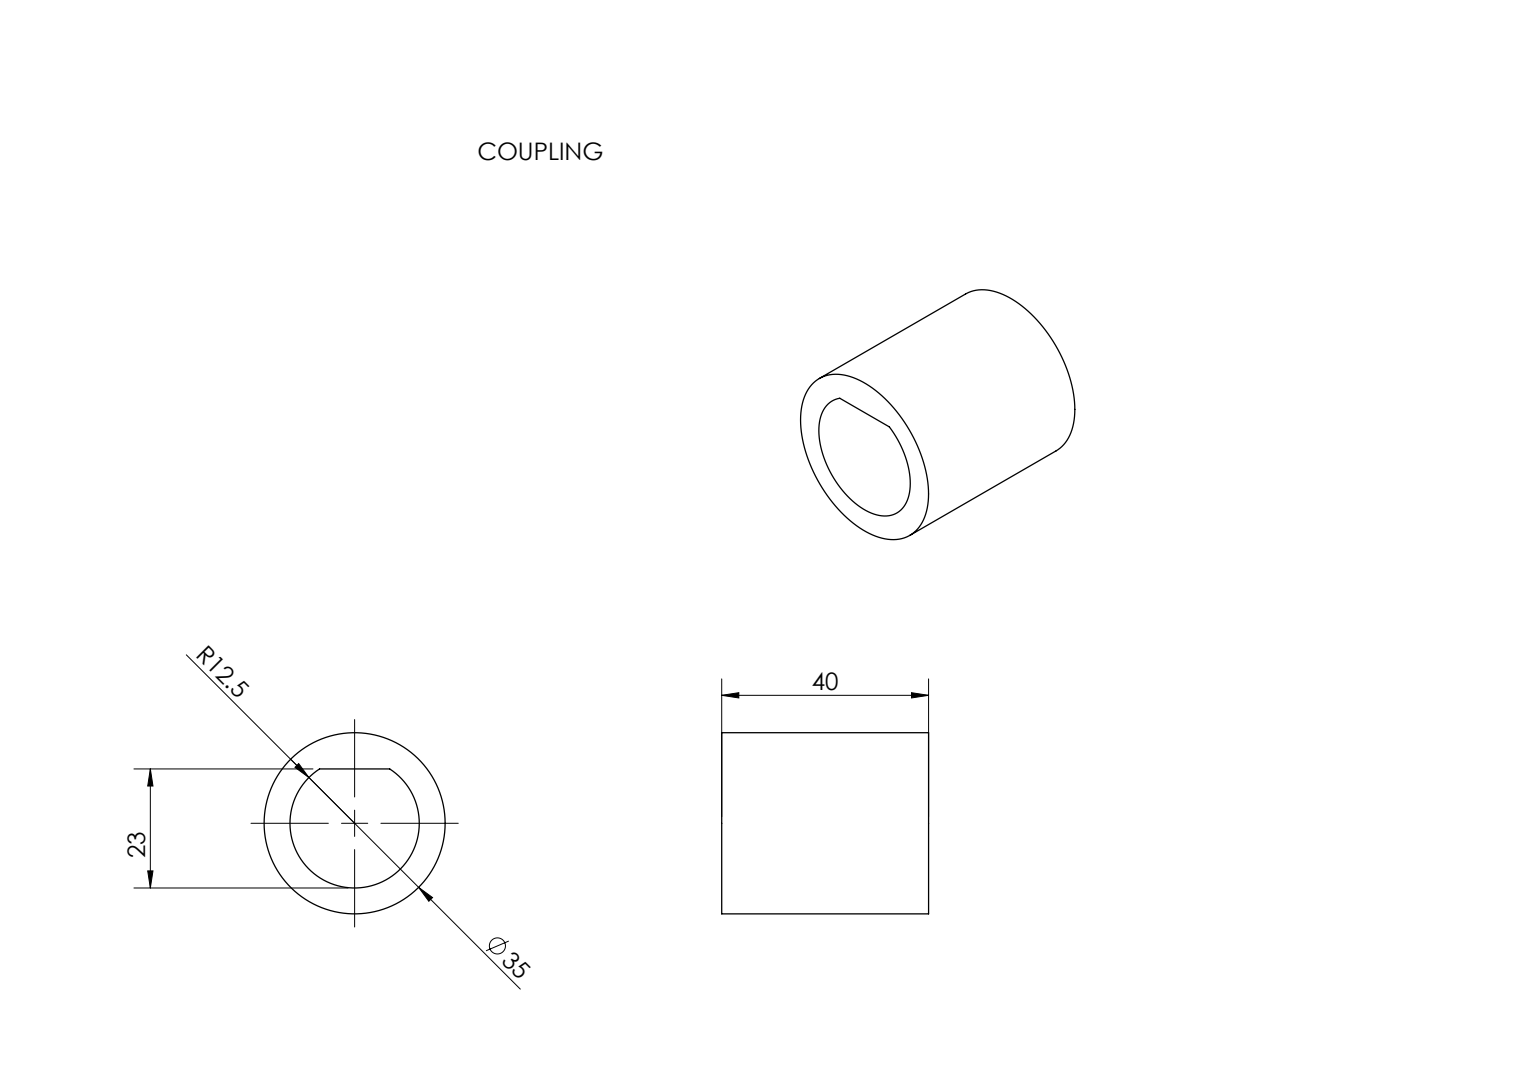
ISO-10303-21;
HEADER;
FILE_DESCRIPTION (('STEP AP214'),
    '1' );
FILE_NAME ('coupling.step',
    '2026-10-08T09:53:37',
    ( '' ),
    ( '' ),
    'SwSTEP 2.0',
    'SolidWorks 2026',
    '' );
FILE_SCHEMA (( 'AUTOMOTIVE_DESIGN' ));
ENDSEC;

DATA;
#136=DIRECTION ( 'NONE',  ( -0.000000000000000000, -0.000000000000000000, -1.000000000000000000 ) ) ;
#689=ORIENTED_EDGE ( 'NONE', *, *, #8488, .T. ) ;
#1357=DIRECTION ( 'NONE',  ( -1.000000000000000000, 0.000000000000000000, 0.000000000000000000 ) ) ;
#1430=AXIS2_PLACEMENT_3D ( 'NONE', #4521, #4148, #32316 ) ;
#1854=EDGE_CURVE ( 'NONE', #52969, #23763, #14079, .T. ) ;
#2181=EDGE_CURVE ( 'NONE', #37253, #52969, #24207, .T. ) ;
#2286=ORIENTED_EDGE ( 'NONE', *, *, #39127, .F. ) ;
#2309=UNCERTAINTY_MEASURE_WITH_UNIT (LENGTH_MEASURE( 1.000000000000000082E-05 ), #36000, 'distance_accuracy_value', 'NONE');
#2430=DIRECTION ( 'NONE',  ( 0.000000000000000000, -1.000000000000000000, 0.000000000000000000 ) ) ;
#2883=FACE_BOUND ( 'NONE', #6394, .T. ) ;
#3015=CARTESIAN_POINT ( 'NONE',  ( 12.49999999999999645, 1.530808498934191127E-15, 20.00000000000000000 ) ) ;
#3992=PRODUCT_DEFINITION_FORMATION_WITH_SPECIFIED_SOURCE ( 'ANY', '', #50605, .NOT_KNOWN. ) ;
#4148=DIRECTION ( 'NONE',  ( 0.000000000000000000, 0.000000000000000000, 1.000000000000000000 ) ) ;
#4234=CIRCLE ( 'NONE', #64274, 12.49999999999999645 ) ;
#4392=DIRECTION ( 'NONE',  ( -1.000000000000000000, 0.000000000000000000, 0.000000000000000000 ) ) ;
#4453=ORIENTED_EDGE ( 'NONE', *, *, #65373, .F. ) ;
#4521=CARTESIAN_POINT ( 'NONE',  ( 0.000000000000000000, 0.000000000000000000, -20.00000000000000000 ) ) ;
#4744=ORIENTED_EDGE ( 'NONE', *, *, #8488, .F. ) ;
#5000=ORIENTED_EDGE ( 'NONE', *, *, #5384, .T. ) ;
#5245=DIRECTION ( 'NONE',  ( 0.000000000000000000, 0.000000000000000000, 1.000000000000000000 ) ) ;
#5273=CARTESIAN_POINT ( 'NONE',  ( -12.49999999999999645, 0.000000000000000000, -20.00000000000000000 ) ) ;
#5384=EDGE_CURVE ( 'NONE', #13441, #37581, #64335, .T. ) ;
#5466=PLANE ( 'NONE',  #40740 ) ;
#5717=CARTESIAN_POINT ( 'NONE',  ( 0.000000000000000000, 0.000000000000000000, -20.00000000000000000 ) ) ;
#6168=CARTESIAN_POINT ( 'NONE',  ( 0.000000000000000000, 0.000000000000000000, 20.00000000000000000 ) ) ;
#6394=EDGE_LOOP ( 'NONE', ( #46540, #31405, #68145, #19160 ) ) ;
#6936=CARTESIAN_POINT ( 'NONE',  ( 6.782329983125270800, 10.49999999999999467, -20.00000000000000000 ) ) ;
#7059=( NAMED_UNIT ( * ) PLANE_ANGLE_UNIT ( ) SI_UNIT ( $, .RADIAN. ) );
#7688=DIRECTION ( 'NONE',  ( 0.000000000000000000, 0.000000000000000000, 1.000000000000000000 ) ) ;
#8488=EDGE_CURVE ( 'NONE', #35321, #37581, #20662, .T. ) ;
#8519=( NAMED_UNIT ( * ) PLANE_ANGLE_UNIT ( ) SI_UNIT ( $, .RADIAN. ) );
#8550=SURFACE_STYLE_FILL_AREA ( #14172 ) ;
#8566=PRODUCT_DEFINITION_CONTEXT ( 'detailed design', #29179, 'design' ) ;
#9214=VECTOR ( 'NONE', #34197, 1000.000000000000000 ) ;
#9241=SHAPE_REPRESENTATION_RELATIONSHIP ( 'NONE' , 'NONE' ,  #15311, #51651 ) ;
#9354=LINE ( 'NONE', #3015, #52898 ) ;
#9498=CARTESIAN_POINT ( 'NONE',  ( 17.50000000000000355, 2.143131898507868643E-15, -20.00000000000000000 ) ) ;
#10144=EDGE_LOOP ( 'NONE', ( #74260, #42905, #52448, #15659 ) ) ;
#10158=AXIS2_PLACEMENT_3D ( 'NONE', #38066, #2430, #54622 ) ;
#10592=CARTESIAN_POINT ( 'NONE',  ( -17.50000000000000355, 0.000000000000000000, 20.00000000000000000 ) ) ;
#11087=DIRECTION ( 'NONE',  ( 0.000000000000000000, 0.000000000000000000, 1.000000000000000000 ) ) ;
#11135=CARTESIAN_POINT ( 'NONE',  ( 0.000000000000000000, 0.000000000000000000, 20.00000000000000000 ) ) ;
#11356=CYLINDRICAL_SURFACE ( 'NONE', #17854, 17.50000000000000355 ) ;
#11556=CARTESIAN_POINT ( 'NONE',  ( 0.000000000000000000, 0.000000000000000000, -20.00000000000000000 ) ) ;
#11695=MECHANICAL_DESIGN_GEOMETRIC_PRESENTATION_REPRESENTATION('',(#51307),#56094);
#12292=VECTOR ( 'NONE', #1357, 1000.000000000000000 ) ;
#12581=LINE ( 'NONE', #6936, #12292 ) ;
#13271=DIRECTION ( 'NONE',  ( -0.000000000000000000, -0.000000000000000000, -1.000000000000000000 ) ) ;
#13441=VERTEX_POINT ( 'NONE', #51685 ) ;
#14079=CIRCLE ( 'NONE', #27275, 12.49999999999999645 ) ;
#14132=SURFACE_STYLE_FILL_AREA ( #20897 ) ;
#14172=FILL_AREA_STYLE ('',( #25830 ) ) ;
#14241=EDGE_CURVE ( 'NONE', #69413, #40595, #58506, .T. ) ;
#14507=ORIENTED_EDGE ( 'NONE', *, *, #41446, .T. ) ;
#14512=FILL_AREA_STYLE_COLOUR ( '', #15948 ) ;
#15189=DIRECTION ( 'NONE',  ( 1.000000000000000000, 0.000000000000000000, 0.000000000000000000 ) ) ;
#15190=ORIENTED_EDGE ( 'NONE', *, *, #23134, .F. ) ;
#15311=SHAPE_REPRESENTATION ( 'coupling', ( #43395 ), #59156 ) ;
#15659=ORIENTED_EDGE ( 'NONE', *, *, #38084, .F. ) ;
#15948=COLOUR_RGB ( '', 0.40784314, 0.44705882, 0.49803922) ;
#16090=EDGE_LOOP ( 'NONE', ( #39134, #689, #64984, #22017 ) ) ;
#16178=CARTESIAN_POINT ( 'NONE',  ( 0.000000000000000000, 0.000000000000000000, 20.00000000000000000 ) ) ;
#16945=ORIENTED_EDGE ( 'NONE', *, *, #47875, .T. ) ;
#16966=DIRECTION ( 'NONE',  ( 0.000000000000000000, 0.000000000000000000, 1.000000000000000000 ) ) ;
#17101=CARTESIAN_POINT ( 'NONE',  ( 0.000000000000000000, 0.000000000000000000, 20.00000000000000000 ) ) ;
#17137=MECHANICAL_DESIGN_GEOMETRIC_PRESENTATION_REPRESENTATION('',(#63986),#41183);
#17739=ORIENTED_EDGE ( 'NONE', *, *, #17822, .T. ) ;
#17822=EDGE_CURVE ( 'NONE', #50481, #37253, #39969, .T. ) ;
#17854=AXIS2_PLACEMENT_3D ( 'NONE', #45962, #136, #69617 ) ;
#17911=CIRCLE ( 'NONE', #59945, 12.49999999999999645 ) ;
#18920=ORIENTED_EDGE ( 'NONE', *, *, #2181, .T. ) ;
#19160=ORIENTED_EDGE ( 'NONE', *, *, #41446, .F. ) ;
#19592=EDGE_LOOP ( 'NONE', ( #15190, #2286, #16945, #17739 ) ) ;
#19735=DIRECTION ( 'NONE',  ( 1.000000000000000000, 0.000000000000000000, 0.000000000000000000 ) ) ;
#20145=( NAMED_UNIT ( * ) PLANE_ANGLE_UNIT ( ) SI_UNIT ( $, .RADIAN. ) );
#20557=FACE_OUTER_BOUND ( 'NONE', #10144, .T. ) ;
#20662=LINE ( 'NONE', #21020, #30170 ) ;
#20831=DIRECTION ( 'NONE',  ( -1.000000000000000000, 0.000000000000000000, 0.000000000000000000 ) ) ;
#20897=FILL_AREA_STYLE ('',( #14512 ) ) ;
#21020=CARTESIAN_POINT ( 'NONE',  ( 17.50000000000000355, 2.143131898507868643E-15, 20.00000000000000000 ) ) ;
#21820=DIRECTION ( 'NONE',  ( 0.000000000000000000, 0.000000000000000000, 1.000000000000000000 ) ) ;
#22017=ORIENTED_EDGE ( 'NONE', *, *, #42840, .F. ) ;
#22325=EDGE_LOOP ( 'NONE', ( #14507, #71175, #36244, #38954 ) ) ;
#22868=CARTESIAN_POINT ( 'NONE',  ( 6.782329983125270800, 10.49999999999999467, 20.00000000000000000 ) ) ;
#22943=EDGE_LOOP ( 'NONE', ( #18920, #29406, #40702, #64202 ) ) ;
#23134=EDGE_CURVE ( 'NONE', #68521, #37253, #12581, .T. ) ;
#23232=DIRECTION ( 'NONE',  ( 1.000000000000000000, 0.000000000000000000, 0.000000000000000000 ) ) ;
#23733=DIRECTION ( 'NONE',  ( 1.000000000000000000, 0.000000000000000000, 0.000000000000000000 ) ) ;
#23763=VERTEX_POINT ( 'NONE', #26423 ) ;
#24207=CIRCLE ( 'NONE', #1430, 12.49999999999999645 ) ;
#24681=PRODUCT_DEFINITION ( 'UNKNOWN', '', #3992, #8566 ) ;
#24741=CARTESIAN_POINT ( 'NONE',  ( 17.50000000000000355, 2.143131898507868643E-15, 20.00000000000000000 ) ) ;
#24976=FACE_OUTER_BOUND ( 'NONE', #50753, .T. ) ;
#25065=CYLINDRICAL_SURFACE ( 'NONE', #40729, 12.49999999999999645 ) ;
#25830=FILL_AREA_STYLE_COLOUR ( '', #40536 ) ;
#26093=AXIS2_PLACEMENT_3D ( 'NONE', #16178, #21820, #27829 ) ;
#26277=FACE_OUTER_BOUND ( 'NONE', #52222, .T. ) ;
#26423=CARTESIAN_POINT ( 'NONE',  ( 12.49999999999999645, 1.530808498934191127E-15, -20.00000000000000000 ) ) ;
#26883=EDGE_LOOP ( 'NONE', ( #4453, #55914, #65318, #59276 ) ) ;
#27219=AXIS2_PLACEMENT_3D ( 'NONE', #70449, #7688, #41531 ) ;
#27275=AXIS2_PLACEMENT_3D ( 'NONE', #5717, #73738, #28621 ) ;
#27829=DIRECTION ( 'NONE',  ( 1.000000000000000000, 0.000000000000000000, 0.000000000000000000 ) ) ;
#28315=LINE ( 'NONE', #72331, #38568 ) ;
#28355=ADVANCED_FACE ( 'NONE', ( #68573 ), #62952, .F. ) ;
#28616=AXIS2_PLACEMENT_3D ( 'NONE', #6168, #40735, #46010 ) ;
#28621=DIRECTION ( 'NONE',  ( 1.000000000000000000, 0.000000000000000000, 0.000000000000000000 ) ) ;
#29179=APPLICATION_CONTEXT ( 'automotive_design' ) ;
#29406=ORIENTED_EDGE ( 'NONE', *, *, #1854, .T. ) ;
#29536=CIRCLE ( 'NONE', #63221, 17.50000000000000355 ) ;
#30170=VECTOR ( 'NONE', #62009, 1000.000000000000000 ) ;
#30186=CARTESIAN_POINT ( 'NONE',  ( -17.50000000000000355, 0.000000000000000000, 20.00000000000000000 ) ) ;
#30547=AXIS2_PLACEMENT_3D ( 'NONE', #39933, #34271, #23733 ) ;
#30679=ORIENTED_EDGE ( 'NONE', *, *, #42840, .T. ) ;
#31405=ORIENTED_EDGE ( 'NONE', *, *, #14241, .F. ) ;
#31438=CARTESIAN_POINT ( 'NONE',  ( 6.782329983125270800, 10.49999999999999467, -20.00000000000000000 ) ) ;
#31919=DIRECTION ( 'NONE',  ( -1.000000000000000000, 0.000000000000000000, 0.000000000000000000 ) ) ;
#32136=ADVANCED_FACE ( 'NONE', ( #54359, #2883 ), #5466, .T. ) ;
#32188=CARTESIAN_POINT ( 'NONE',  ( 0.000000000000000000, 0.000000000000000000, 20.00000000000000000 ) ) ;
#32316=DIRECTION ( 'NONE',  ( 1.000000000000000000, 0.000000000000000000, 0.000000000000000000 ) ) ;
#32777=ADVANCED_FACE ( 'NONE', ( #51949 ), #11356, .T. ) ;
#34060=DIRECTION ( 'NONE',  ( -0.000000000000000000, -0.000000000000000000, -1.000000000000000000 ) ) ;
#34197=DIRECTION ( 'NONE',  ( -0.000000000000000000, -0.000000000000000000, -1.000000000000000000 ) ) ;
#34271=DIRECTION ( 'NONE',  ( 0.000000000000000000, 0.000000000000000000, 1.000000000000000000 ) ) ;
#35321=VERTEX_POINT ( 'NONE', #24741 ) ;
#35624=SURFACE_SIDE_STYLE ('',( #8550 ) ) ;
#36000=( LENGTH_UNIT ( ) NAMED_UNIT ( * ) SI_UNIT ( .MILLI., .METRE. ) );
#36192=DIRECTION ( 'NONE',  ( 1.000000000000000000, 0.000000000000000000, 0.000000000000000000 ) ) ;
#36244=ORIENTED_EDGE ( 'NONE', *, *, #2181, .F. ) ;
#36257=FACE_BOUND ( 'NONE', #22943, .T. ) ;
#36710=CARTESIAN_POINT ( 'NONE',  ( 0.000000000000000000, 0.000000000000000000, 20.00000000000000000 ) ) ;
#36733=PRODUCT_DEFINITION_SHAPE ( 'NONE', 'NONE',  #24681 ) ;
#37084=SURFACE_STYLE_USAGE ( .BOTH. , #54014 ) ;
#37111=DIRECTION ( 'NONE',  ( -0.000000000000000000, -0.000000000000000000, -1.000000000000000000 ) ) ;
#37253=VERTEX_POINT ( 'NONE', #74224 ) ;
#37581=VERTEX_POINT ( 'NONE', #9498 ) ;
#37592=CARTESIAN_POINT ( 'NONE',  ( -12.49999999999999645, 0.000000000000000000, 20.00000000000000000 ) ) ;
#38066=CARTESIAN_POINT ( 'NONE',  ( 6.782329983125270800, 10.49999999999999467, 20.00000000000000000 ) ) ;
#38084=EDGE_CURVE ( 'NONE', #49570, #52969, #62802, .T. ) ;
#38188=( LENGTH_UNIT ( ) NAMED_UNIT ( * ) SI_UNIT ( .MILLI., .METRE. ) );
#38212=CYLINDRICAL_SURFACE ( 'NONE', #71933, 12.49999999999999645 ) ;
#38321=CARTESIAN_POINT ( 'NONE',  ( 0.000000000000000000, 0.000000000000000000, 20.00000000000000000 ) ) ;
#38473=ORIENTED_EDGE ( 'NONE', *, *, #39207, .T. ) ;
#38568=VECTOR ( 'NONE', #20831, 1000.000000000000000 ) ;
#38954=ORIENTED_EDGE ( 'NONE', *, *, #17822, .F. ) ;
#39127=EDGE_CURVE ( 'NONE', #40595, #68521, #68712, .T. ) ;
#39134=ORIENTED_EDGE ( 'NONE', *, *, #66536, .F. ) ;
#39207=EDGE_CURVE ( 'NONE', #44003, #35321, #41733, .T. ) ;
#39393=CARTESIAN_POINT ( 'NONE',  ( 0.000000000000000000, 0.000000000000000000, 20.00000000000000000 ) ) ;
#39719=CYLINDRICAL_SURFACE ( 'NONE', #41983, 17.50000000000000355 ) ;
#39750=APPLICATION_CONTEXT ( 'automotive_design' ) ;
#39933=CARTESIAN_POINT ( 'NONE',  ( 0.000000000000000000, 0.000000000000000000, -20.00000000000000000 ) ) ;
#39969=LINE ( 'NONE', #62924, #71335 ) ;
#40536=COLOUR_RGB ( '', 0.40784314, 0.44705882, 0.49803922) ;
#40586=EDGE_CURVE ( 'NONE', #23763, #68521, #17911, .T. ) ;
#40595=VERTEX_POINT ( 'NONE', #22868 ) ;
#40702=ORIENTED_EDGE ( 'NONE', *, *, #40586, .T. ) ;
#40729=AXIS2_PLACEMENT_3D ( 'NONE', #36710, #42366, #46903 ) ;
#40734=DIRECTION ( 'NONE',  ( 0.000000000000000000, 0.000000000000000000, 1.000000000000000000 ) ) ;
#40735=DIRECTION ( 'NONE',  ( -0.000000000000000000, -0.000000000000000000, -1.000000000000000000 ) ) ;
#40740=AXIS2_PLACEMENT_3D ( 'NONE', #17101, #11087, #73854 ) ;
#40748=ADVANCED_FACE ( 'NONE', ( #52906 ), #25065, .F. ) ;
#40922=ADVANCED_FACE ( 'NONE', ( #20557 ), #38212, .F. ) ;
#41183=( GEOMETRIC_REPRESENTATION_CONTEXT ( 3 ) GLOBAL_UNCERTAINTY_ASSIGNED_CONTEXT ( ( #65621 ) ) GLOBAL_UNIT_ASSIGNED_CONTEXT ( ( #38188, #8519, #48726 ) ) REPRESENTATION_CONTEXT ( 'NONE', 'WORKASPACE' ) );
#41446=EDGE_CURVE ( 'NONE', #50481, #49570, #71877, .T. ) ;
#41531=DIRECTION ( 'NONE',  ( 1.000000000000000000, 0.000000000000000000, -0.000000000000000000 ) ) ;
#41733=CIRCLE ( 'NONE', #44096, 17.50000000000000355 ) ;
#41983=AXIS2_PLACEMENT_3D ( 'NONE', #11135, #34060, #31919 ) ;
#42028=PRESENTATION_STYLE_ASSIGNMENT (( #48029 ) ) ;
#42366=DIRECTION ( 'NONE',  ( -0.000000000000000000, -0.000000000000000000, -1.000000000000000000 ) ) ;
#42840=EDGE_CURVE ( 'NONE', #44003, #13441, #58775, .T. ) ;
#42905=ORIENTED_EDGE ( 'NONE', *, *, #65373, .T. ) ;
#43039=CARTESIAN_POINT ( 'NONE',  ( 0.000000000000000000, 0.000000000000000000, 20.00000000000000000 ) ) ;
#43063=UNCERTAINTY_MEASURE_WITH_UNIT (LENGTH_MEASURE( 1.000000000000000082E-05 ), #64548, 'distance_accuracy_value', 'NONE');
#43395=AXIS2_PLACEMENT_3D ( 'NONE', #48320, #71232, #19735 ) ;
#43941=AXIS2_PLACEMENT_3D ( 'NONE', #46372, #40734, #36192 ) ;
#44003=VERTEX_POINT ( 'NONE', #10592 ) ;
#44096=AXIS2_PLACEMENT_3D ( 'NONE', #39393, #55932, #67587 ) ;
#45962=CARTESIAN_POINT ( 'NONE',  ( 0.000000000000000000, 0.000000000000000000, 20.00000000000000000 ) ) ;
#46010=DIRECTION ( 'NONE',  ( -1.000000000000000000, 0.000000000000000000, 0.000000000000000000 ) ) ;
#46372=CARTESIAN_POINT ( 'NONE',  ( 0.000000000000000000, 0.000000000000000000, -20.00000000000000000 ) ) ;
#46512=VECTOR ( 'NONE', #56312, 1000.000000000000000 ) ;
#46540=ORIENTED_EDGE ( 'NONE', *, *, #47875, .F. ) ;
#46758=CARTESIAN_POINT ( 'NONE',  ( 12.49999999999999645, 1.530808498934191127E-15, 20.00000000000000000 ) ) ;
#46903=DIRECTION ( 'NONE',  ( -1.000000000000000000, 0.000000000000000000, 0.000000000000000000 ) ) ;
#47875=EDGE_CURVE ( 'NONE', #40595, #50481, #28315, .T. ) ;
#48029=SURFACE_STYLE_USAGE ( .BOTH. , #35624 ) ;
#48320=CARTESIAN_POINT ( 'NONE',  ( 0.000000000000000000, 0.000000000000000000, 0.000000000000000000 ) ) ;
#48519=ORIENTED_EDGE ( 'NONE', *, *, #52548, .F. ) ;
#48726=( NAMED_UNIT ( * ) SI_UNIT ( $, .STERADIAN. ) SOLID_ANGLE_UNIT ( ) );
#49279=EDGE_LOOP ( 'NONE', ( #38473, #65303 ) ) ;
#49570=VERTEX_POINT ( 'NONE', #37592 ) ;
#49701=FACE_OUTER_BOUND ( 'NONE', #19592, .T. ) ;
#50481=VERTEX_POINT ( 'NONE', #64881 ) ;
#50605=PRODUCT ( 'coupling', 'coupling', '', ( #67417 ) ) ;
#50753=EDGE_LOOP ( 'NONE', ( #55966, #48519 ) ) ;
#51081=DIRECTION ( 'NONE',  ( 1.000000000000000000, 0.000000000000000000, 0.000000000000000000 ) ) ;
#51307=STYLED_ITEM ( 'NONE', ( #42028 ), #61761 ) ;
#51412=DIRECTION ( 'NONE',  ( 0.000000000000000000, 0.000000000000000000, 1.000000000000000000 ) ) ;
#51651=ADVANCED_BREP_SHAPE_REPRESENTATION ( '', ( #61761, #43395 ), #59156 ) ;
#51685=CARTESIAN_POINT ( 'NONE',  ( -17.50000000000000355, 0.000000000000000000, -20.00000000000000000 ) ) ;
#51949=FACE_OUTER_BOUND ( 'NONE', #16090, .T. ) ;
#52222=EDGE_LOOP ( 'NONE', ( #4744, #64257, #30679, #5000 ) ) ;
#52448=ORIENTED_EDGE ( 'NONE', *, *, #1854, .F. ) ;
#52548=EDGE_CURVE ( 'NONE', #37581, #13441, #62998, .T. ) ;
#52575=VECTOR ( 'NONE', #13271, 1000.000000000000000 ) ;
#52898=VECTOR ( 'NONE', #66513, 1000.000000000000000 ) ;
#52906=FACE_OUTER_BOUND ( 'NONE', #26883, .T. ) ;
#52969=VERTEX_POINT ( 'NONE', #5273 ) ;
#54014=SURFACE_SIDE_STYLE ('',( #14132 ) ) ;
#54359=FACE_OUTER_BOUND ( 'NONE', #49279, .T. ) ;
#54622=DIRECTION ( 'NONE',  ( 0.000000000000000000, -0.000000000000000000, -1.000000000000000000 ) ) ;
#54741=( NAMED_UNIT ( * ) SI_UNIT ( $, .STERADIAN. ) SOLID_ANGLE_UNIT ( ) );
#55255=AXIS2_PLACEMENT_3D ( 'NONE', #43039, #66702, #15189 ) ;
#55914=ORIENTED_EDGE ( 'NONE', *, *, #14241, .T. ) ;
#55932=DIRECTION ( 'NONE',  ( 0.000000000000000000, 0.000000000000000000, 1.000000000000000000 ) ) ;
#55966=ORIENTED_EDGE ( 'NONE', *, *, #5384, .F. ) ;
#56094=( GEOMETRIC_REPRESENTATION_CONTEXT ( 3 ) GLOBAL_UNCERTAINTY_ASSIGNED_CONTEXT ( ( #2309 ) ) GLOBAL_UNIT_ASSIGNED_CONTEXT ( ( #36000, #7059, #65329 ) ) REPRESENTATION_CONTEXT ( 'NONE', 'WORKASPACE' ) );
#56312=DIRECTION ( 'NONE',  ( -0.000000000000000000, -0.000000000000000000, -1.000000000000000000 ) ) ;
#56522=SHAPE_DEFINITION_REPRESENTATION ( #36733, #15311 ) ;
#56688=CARTESIAN_POINT ( 'NONE',  ( 6.782329983125270800, 10.49999999999999467, 20.00000000000000000 ) ) ;
#57862=ADVANCED_FACE ( 'NONE', ( #49701 ), #66999, .T. ) ;
#57994=DIRECTION ( 'NONE',  ( -0.000000000000000000, -0.000000000000000000, -1.000000000000000000 ) ) ;
#58506=CIRCLE ( 'NONE', #26093, 12.49999999999999645 ) ;
#58775=LINE ( 'NONE', #30186, #52575 ) ;
#59156=( GEOMETRIC_REPRESENTATION_CONTEXT ( 3 ) GLOBAL_UNCERTAINTY_ASSIGNED_CONTEXT ( ( #43063 ) ) GLOBAL_UNIT_ASSIGNED_CONTEXT ( ( #64548, #20145, #54741 ) ) REPRESENTATION_CONTEXT ( 'NONE', 'WORKASPACE' ) );
#59276=ORIENTED_EDGE ( 'NONE', *, *, #40586, .F. ) ;
#59945=AXIS2_PLACEMENT_3D ( 'NONE', #11556, #51412, #23232 ) ;
#60035=PRESENTATION_STYLE_ASSIGNMENT (( #37084 ) ) ;
#61761=MANIFOLD_SOLID_BREP ( 'Boss-Extrude1', #62005 ) ;
#62005=CLOSED_SHELL ( 'NONE', ( #40922, #28355, #32777, #32136, #68758, #64035, #40748, #57862 ) ) ;
#62009=DIRECTION ( 'NONE',  ( -0.000000000000000000, -0.000000000000000000, -1.000000000000000000 ) ) ;
#62802=LINE ( 'NONE', #67299, #9214 ) ;
#62924=CARTESIAN_POINT ( 'NONE',  ( -6.782329983125270800, 10.49999999999999467, 20.00000000000000000 ) ) ;
#62952=CYLINDRICAL_SURFACE ( 'NONE', #28616, 12.49999999999999645 ) ;
#62998=CIRCLE ( 'NONE', #30547, 17.50000000000000355 ) ;
#63221=AXIS2_PLACEMENT_3D ( 'NONE', #74094, #16966, #69574 ) ;
#63986=STYLED_ITEM ( 'NONE', ( #60035 ), #51651 ) ;
#64035=ADVANCED_FACE ( 'NONE', ( #26277 ), #39719, .T. ) ;
#64202=ORIENTED_EDGE ( 'NONE', *, *, #23134, .T. ) ;
#64257=ORIENTED_EDGE ( 'NONE', *, *, #39207, .F. ) ;
#64274=AXIS2_PLACEMENT_3D ( 'NONE', #38321, #5245, #51081 ) ;
#64335=CIRCLE ( 'NONE', #43941, 17.50000000000000355 ) ;
#64548=( LENGTH_UNIT ( ) NAMED_UNIT ( * ) SI_UNIT ( .MILLI., .METRE. ) );
#64845=PLANE ( 'NONE',  #27219 ) ;
#64881=CARTESIAN_POINT ( 'NONE',  ( -6.782329983125270800, 10.49999999999999467, 20.00000000000000000 ) ) ;
#64984=ORIENTED_EDGE ( 'NONE', *, *, #52548, .T. ) ;
#65303=ORIENTED_EDGE ( 'NONE', *, *, #66536, .T. ) ;
#65318=ORIENTED_EDGE ( 'NONE', *, *, #39127, .T. ) ;
#65329=( NAMED_UNIT ( * ) SI_UNIT ( $, .STERADIAN. ) SOLID_ANGLE_UNIT ( ) );
#65373=EDGE_CURVE ( 'NONE', #69413, #23763, #9354, .T. ) ;
#65621=UNCERTAINTY_MEASURE_WITH_UNIT (LENGTH_MEASURE( 1.000000000000000082E-05 ), #38188, 'distance_accuracy_value', 'NONE');
#66513=DIRECTION ( 'NONE',  ( -0.000000000000000000, -0.000000000000000000, -1.000000000000000000 ) ) ;
#66536=EDGE_CURVE ( 'NONE', #35321, #44003, #29536, .T. ) ;
#66702=DIRECTION ( 'NONE',  ( 0.000000000000000000, 0.000000000000000000, 1.000000000000000000 ) ) ;
#66949=EDGE_CURVE ( 'NONE', #49570, #69413, #4234, .T. ) ;
#66999=PLANE ( 'NONE',  #10158 ) ;
#67299=CARTESIAN_POINT ( 'NONE',  ( -12.49999999999999645, 0.000000000000000000, 20.00000000000000000 ) ) ;
#67417=PRODUCT_CONTEXT ( 'NONE', #39750, 'mechanical' ) ;
#67587=DIRECTION ( 'NONE',  ( 1.000000000000000000, 0.000000000000000000, 0.000000000000000000 ) ) ;
#68145=ORIENTED_EDGE ( 'NONE', *, *, #66949, .F. ) ;
#68521=VERTEX_POINT ( 'NONE', #31438 ) ;
#68573=FACE_OUTER_BOUND ( 'NONE', #22325, .T. ) ;
#68712=LINE ( 'NONE', #56688, #46512 ) ;
#68758=ADVANCED_FACE ( 'NONE', ( #24976, #36257 ), #64845, .F. ) ;
#69413=VERTEX_POINT ( 'NONE', #46758 ) ;
#69574=DIRECTION ( 'NONE',  ( 1.000000000000000000, 0.000000000000000000, 0.000000000000000000 ) ) ;
#69617=DIRECTION ( 'NONE',  ( -1.000000000000000000, 0.000000000000000000, 0.000000000000000000 ) ) ;
#70449=CARTESIAN_POINT ( 'NONE',  ( 0.000000000000000000, 0.000000000000000000, -20.00000000000000000 ) ) ;
#71175=ORIENTED_EDGE ( 'NONE', *, *, #38084, .T. ) ;
#71232=DIRECTION ( 'NONE',  ( 0.000000000000000000, 0.000000000000000000, 1.000000000000000000 ) ) ;
#71335=VECTOR ( 'NONE', #57994, 1000.000000000000000 ) ;
#71877=CIRCLE ( 'NONE', #55255, 12.49999999999999645 ) ;
#71933=AXIS2_PLACEMENT_3D ( 'NONE', #32188, #37111, #4392 ) ;
#72331=CARTESIAN_POINT ( 'NONE',  ( 6.782329983125270800, 10.49999999999999467, 20.00000000000000000 ) ) ;
#73738=DIRECTION ( 'NONE',  ( 0.000000000000000000, 0.000000000000000000, 1.000000000000000000 ) ) ;
#73854=DIRECTION ( 'NONE',  ( 1.000000000000000000, 0.000000000000000000, -0.000000000000000000 ) ) ;
#74094=CARTESIAN_POINT ( 'NONE',  ( 0.000000000000000000, 0.000000000000000000, 20.00000000000000000 ) ) ;
#74224=CARTESIAN_POINT ( 'NONE',  ( -6.782329983125270800, 10.49999999999999467, -20.00000000000000000 ) ) ;
#74260=ORIENTED_EDGE ( 'NONE', *, *, #66949, .T. ) ;
ENDSEC;
END-ISO-10303-21;
